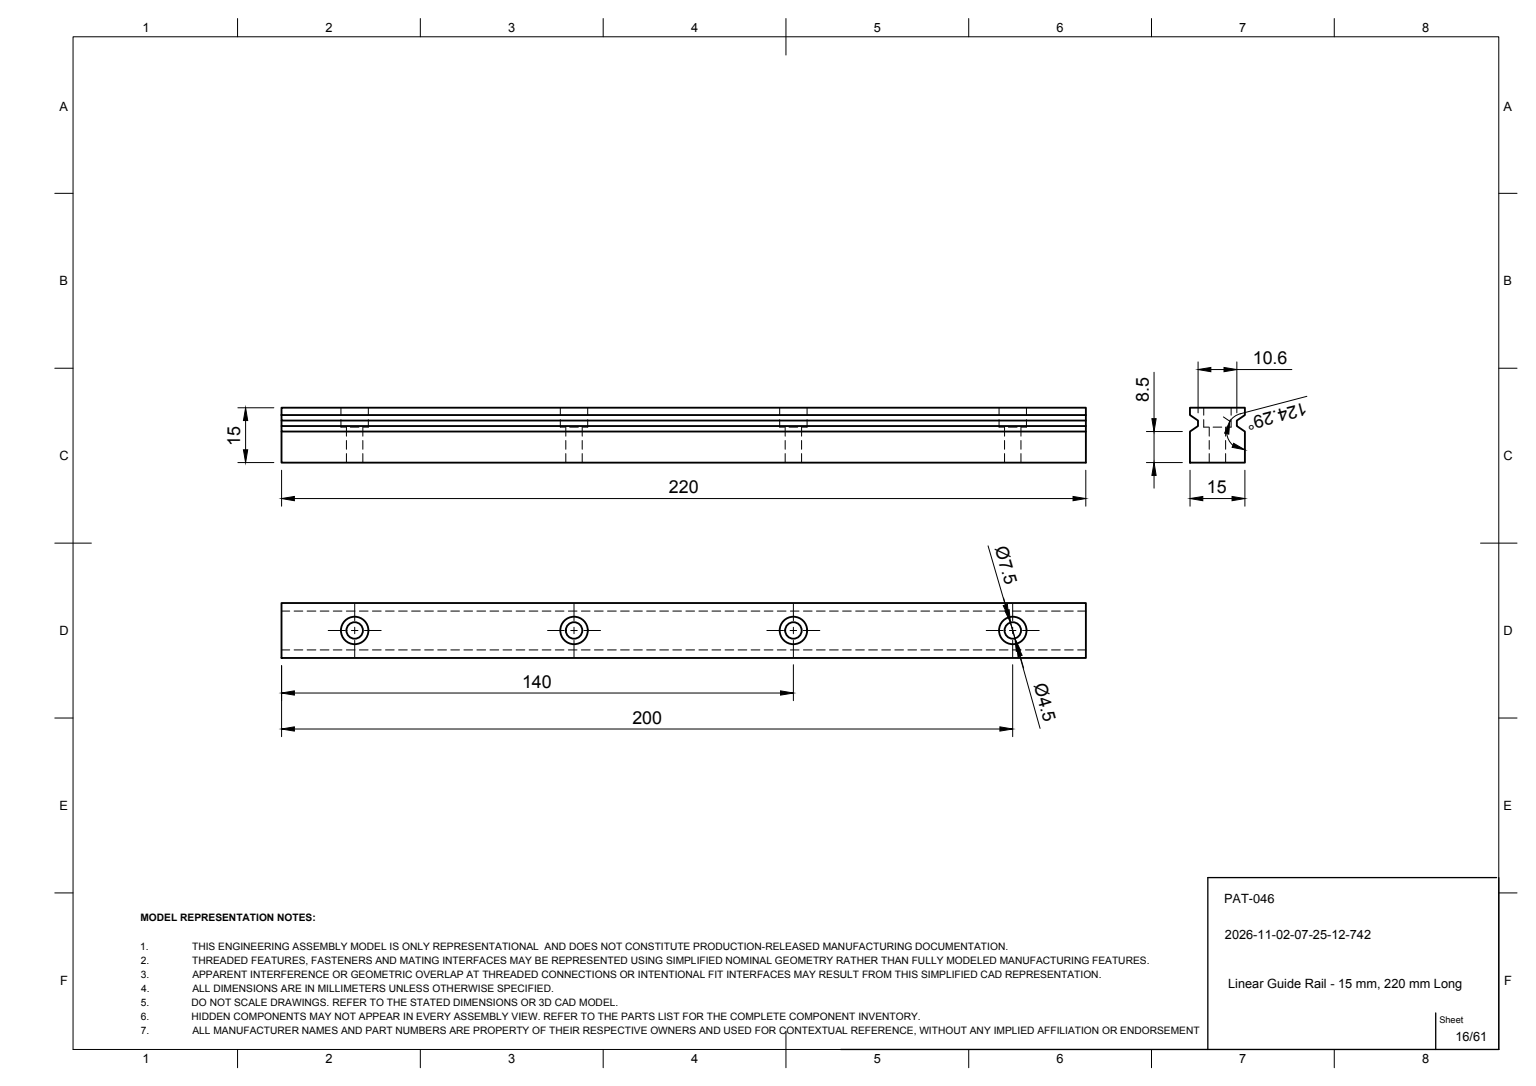
ISO-10303-21;
HEADER;
/* Generated by software containing ST-Developer
 * from STEP Tools, Inc. (www.steptools.com) 
 */

FILE_DESCRIPTION(
/* description */ ('Gear mesh backlash fixture'),
/* implementation_level */ '2;1');

FILE_NAME(
/* name */ 'Linear Guide Rail - 15 mm, 220 mm Long.step',
/* time_stamp */ '2026-10-28T03:26:00-07:00',
/* author */ (''),
/* organization */ (''),
/* preprocessor_version */ 'ST-DEVELOPER v20.2',
/* originating_system */ 'Autodesk Translation Framework v15.17.0.0',
/* authorisation */ '');

FILE_SCHEMA (('AUTOMOTIVE_DESIGN { 1 0 10303 214 3 1 1 }'));
ENDSEC;

DATA;
#10=MECHANICAL_DESIGN_GEOMETRIC_PRESENTATION_REPRESENTATION('',(#1027),#57900);
#927=SHAPE_REPRESENTATION_RELATIONSHIP('SRR','None',#58122,#977);
#977=ADVANCED_BREP_SHAPE_REPRESENTATION('',(#1092),#57855);
#1027=STYLED_ITEM('',(#58458),#1092);
#1092=MANIFOLD_SOLID_BREP('Body1',#13587);
#1205=FACE_BOUND('',#2643,.T.);
#1206=FACE_BOUND('',#2646,.T.);
#1207=FACE_BOUND('',#2649,.T.);
#1208=FACE_BOUND('',#2652,.T.);
#1209=FACE_BOUND('',#2662,.T.);
#1210=FACE_BOUND('',#2663,.T.);
#1211=FACE_BOUND('',#2664,.T.);
#1212=FACE_BOUND('',#2665,.T.);
#1213=FACE_BOUND('',#2672,.T.);
#1214=FACE_BOUND('',#2673,.T.);
#1215=FACE_BOUND('',#2674,.T.);
#1216=FACE_BOUND('',#2675,.T.);
#1395=PLANE('',#14457);
#1396=PLANE('',#14462);
#1397=PLANE('',#14467);
#1398=PLANE('',#14472);
#1399=PLANE('',#14482);
#1400=PLANE('',#14483);
#1401=PLANE('',#14484);
#1402=PLANE('',#14485);
#1403=PLANE('',#14486);
#1404=PLANE('',#14487);
#1405=PLANE('',#14488);
#1406=PLANE('',#14489);
#1407=PLANE('',#14490);
#1408=PLANE('',#14491);
#1409=PLANE('',#14492);
#1410=PLANE('',#14493);
#1411=PLANE('',#14494);
#1412=PLANE('',#14495);
#1814=FACE_OUTER_BOUND('',#2641,.T.);
#1815=FACE_OUTER_BOUND('',#2642,.T.);
#1816=FACE_OUTER_BOUND('',#2644,.T.);
#1817=FACE_OUTER_BOUND('',#2645,.T.);
#1818=FACE_OUTER_BOUND('',#2647,.T.);
#1819=FACE_OUTER_BOUND('',#2648,.T.);
#1820=FACE_OUTER_BOUND('',#2650,.T.);
#1821=FACE_OUTER_BOUND('',#2651,.T.);
#1822=FACE_OUTER_BOUND('',#2653,.T.);
#1823=FACE_OUTER_BOUND('',#2654,.T.);
#1824=FACE_OUTER_BOUND('',#2655,.T.);
#1825=FACE_OUTER_BOUND('',#2656,.T.);
#1826=FACE_OUTER_BOUND('',#2657,.T.);
#1827=FACE_OUTER_BOUND('',#2658,.T.);
#1828=FACE_OUTER_BOUND('',#2659,.T.);
#1829=FACE_OUTER_BOUND('',#2660,.T.);
#1830=FACE_OUTER_BOUND('',#2661,.T.);
#1831=FACE_OUTER_BOUND('',#2666,.T.);
#1832=FACE_OUTER_BOUND('',#2667,.T.);
#1833=FACE_OUTER_BOUND('',#2668,.T.);
#1834=FACE_OUTER_BOUND('',#2669,.T.);
#1835=FACE_OUTER_BOUND('',#2670,.T.);
#1836=FACE_OUTER_BOUND('',#2671,.T.);
#1837=FACE_OUTER_BOUND('',#2676,.T.);
#1838=FACE_OUTER_BOUND('',#2677,.T.);
#1839=FACE_OUTER_BOUND('',#2678,.T.);
#2641=EDGE_LOOP('',(#9427,#9428,#9429,#9430));
#2642=EDGE_LOOP('',(#9431));
#2643=EDGE_LOOP('',(#9432));
#2644=EDGE_LOOP('',(#9433,#9434,#9435,#9436));
#2645=EDGE_LOOP('',(#9437));
#2646=EDGE_LOOP('',(#9438));
#2647=EDGE_LOOP('',(#9439,#9440,#9441,#9442));
#2648=EDGE_LOOP('',(#9443));
#2649=EDGE_LOOP('',(#9444));
#2650=EDGE_LOOP('',(#9445,#9446,#9447,#9448));
#2651=EDGE_LOOP('',(#9449));
#2652=EDGE_LOOP('',(#9450));
#2653=EDGE_LOOP('',(#9451,#9452,#9453,#9454));
#2654=EDGE_LOOP('',(#9455,#9456,#9457,#9458));
#2655=EDGE_LOOP('',(#9459,#9460,#9461,#9462));
#2656=EDGE_LOOP('',(#9463,#9464,#9465,#9466));
#2657=EDGE_LOOP('',(#9467,#9468,#9469,#9470));
#2658=EDGE_LOOP('',(#9471,#9472,#9473,#9474));
#2659=EDGE_LOOP('',(#9475,#9476,#9477,#9478));
#2660=EDGE_LOOP('',(#9479,#9480,#9481,#9482));
#2661=EDGE_LOOP('',(#9483,#9484,#9485,#9486));
#2662=EDGE_LOOP('',(#9487));
#2663=EDGE_LOOP('',(#9488));
#2664=EDGE_LOOP('',(#9489));
#2665=EDGE_LOOP('',(#9490));
#2666=EDGE_LOOP('',(#9491,#9492,#9493,#9494));
#2667=EDGE_LOOP('',(#9495,#9496,#9497,#9498));
#2668=EDGE_LOOP('',(#9499,#9500,#9501,#9502));
#2669=EDGE_LOOP('',(#9503,#9504,#9505,#9506));
#2670=EDGE_LOOP('',(#9507,#9508,#9509,#9510));
#2671=EDGE_LOOP('',(#9511,#9512,#9513,#9514));
#2672=EDGE_LOOP('',(#9515));
#2673=EDGE_LOOP('',(#9516));
#2674=EDGE_LOOP('',(#9517));
#2675=EDGE_LOOP('',(#9518));
#2676=EDGE_LOOP('',(#9519,#9520,#9521,#9522));
#2677=EDGE_LOOP('',(#9523,#9524,#9525,#9526,#9527,#9528,#9529,#9530,#9531,
#9532,#9533,#9534));
#2678=EDGE_LOOP('',(#9535,#9536,#9537,#9538,#9539,#9540,#9541,#9542,#9543,
#9544,#9545,#9546));
#3553=LINE('',#19918,#4442);
#3554=LINE('',#19927,#4443);
#3555=LINE('',#19936,#4444);
#3556=LINE('',#19945,#4445);
#3557=LINE('',#19953,#4446);
#3558=LINE('',#19957,#4447);
#3559=LINE('',#19961,#4448);
#3560=LINE('',#19965,#4449);
#3561=LINE('',#19969,#4450);
#3562=LINE('',#19971,#4451);
#3563=LINE('',#19973,#4452);
#3564=LINE('',#19974,#4453);
#3565=LINE('',#19977,#4454);
#3566=LINE('',#19979,#4455);
#3567=LINE('',#19980,#4456);
#3568=LINE('',#19983,#4457);
#3569=LINE('',#19985,#4458);
#3570=LINE('',#19986,#4459);
#3571=LINE('',#19989,#4460);
#3572=LINE('',#19991,#4461);
#3573=LINE('',#19992,#4462);
#3574=LINE('',#19995,#4463);
#3575=LINE('',#19997,#4464);
#3576=LINE('',#19998,#4465);
#3577=LINE('',#20001,#4466);
#3578=LINE('',#20003,#4467);
#3579=LINE('',#20004,#4468);
#3580=LINE('',#20007,#4469);
#3581=LINE('',#20009,#4470);
#3582=LINE('',#20010,#4471);
#3583=LINE('',#20013,#4472);
#3584=LINE('',#20015,#4473);
#3585=LINE('',#20016,#4474);
#3586=LINE('',#20019,#4475);
#3587=LINE('',#20021,#4476);
#3588=LINE('',#20022,#4477);
#3589=LINE('',#20025,#4478);
#3590=LINE('',#20027,#4479);
#3591=LINE('',#20028,#4480);
#3592=LINE('',#20031,#4481);
#3593=LINE('',#20033,#4482);
#3594=LINE('',#20034,#4483);
#3595=LINE('',#20036,#4484);
#3596=LINE('',#20037,#4485);
#4442=VECTOR('',#16242,0.375);
#4443=VECTOR('',#16253,0.375);
#4444=VECTOR('',#16264,0.375);
#4445=VECTOR('',#16275,0.375);
#4446=VECTOR('',#16286,0.225);
#4447=VECTOR('',#16291,0.225);
#4448=VECTOR('',#16296,0.225);
#4449=VECTOR('',#16301,0.225000000000001);
#4450=VECTOR('',#16304,1.);
#4451=VECTOR('',#16305,1.);
#4452=VECTOR('',#16306,1.);
#4453=VECTOR('',#16307,1.);
#4454=VECTOR('',#16310,1.);
#4455=VECTOR('',#16311,1.);
#4456=VECTOR('',#16312,1.);
#4457=VECTOR('',#16315,1.);
#4458=VECTOR('',#16316,1.);
#4459=VECTOR('',#16317,1.);
#4460=VECTOR('',#16320,1.);
#4461=VECTOR('',#16321,1.);
#4462=VECTOR('',#16322,1.);
#4463=VECTOR('',#16325,1.);
#4464=VECTOR('',#16326,1.);
#4465=VECTOR('',#16327,1.);
#4466=VECTOR('',#16330,1.);
#4467=VECTOR('',#16331,1.);
#4468=VECTOR('',#16332,1.);
#4469=VECTOR('',#16335,1.);
#4470=VECTOR('',#16336,1.);
#4471=VECTOR('',#16337,1.);
#4472=VECTOR('',#16340,1.);
#4473=VECTOR('',#16341,1.);
#4474=VECTOR('',#16342,1.);
#4475=VECTOR('',#16345,1.);
#4476=VECTOR('',#16346,1.);
#4477=VECTOR('',#16347,1.);
#4478=VECTOR('',#16350,1.);
#4479=VECTOR('',#16351,1.);
#4480=VECTOR('',#16352,1.);
#4481=VECTOR('',#16355,1.);
#4482=VECTOR('',#16356,1.);
#4483=VECTOR('',#16357,1.);
#4484=VECTOR('',#16360,1.);
#4485=VECTOR('',#16361,1.);
#5314=CIRCLE('',#14455,0.375);
#5315=CIRCLE('',#14456,0.375);
#5316=CIRCLE('',#14458,0.225);
#5317=CIRCLE('',#14460,0.375);
#5318=CIRCLE('',#14461,0.375);
#5319=CIRCLE('',#14463,0.225);
#5320=CIRCLE('',#14465,0.375);
#5321=CIRCLE('',#14466,0.375);
#5322=CIRCLE('',#14468,0.225);
#5323=CIRCLE('',#14470,0.375);
#5324=CIRCLE('',#14471,0.375);
#5325=CIRCLE('',#14473,0.225000000000001);
#5326=CIRCLE('',#14475,0.225);
#5327=CIRCLE('',#14477,0.225);
#5328=CIRCLE('',#14479,0.225);
#5329=CIRCLE('',#14481,0.225000000000001);
#5959=VERTEX_POINT('',#19915);
#5960=VERTEX_POINT('',#19917);
#5961=VERTEX_POINT('',#19921);
#5962=VERTEX_POINT('',#19924);
#5963=VERTEX_POINT('',#19926);
#5964=VERTEX_POINT('',#19930);
#5965=VERTEX_POINT('',#19933);
#5966=VERTEX_POINT('',#19935);
#5967=VERTEX_POINT('',#19939);
#5968=VERTEX_POINT('',#19942);
#5969=VERTEX_POINT('',#19944);
#5970=VERTEX_POINT('',#19948);
#5971=VERTEX_POINT('',#19951);
#5972=VERTEX_POINT('',#19955);
#5973=VERTEX_POINT('',#19959);
#5974=VERTEX_POINT('',#19963);
#5975=VERTEX_POINT('',#19967);
#5976=VERTEX_POINT('',#19968);
#5977=VERTEX_POINT('',#19970);
#5978=VERTEX_POINT('',#19972);
#5979=VERTEX_POINT('',#19976);
#5980=VERTEX_POINT('',#19978);
#5981=VERTEX_POINT('',#19982);
#5982=VERTEX_POINT('',#19984);
#5983=VERTEX_POINT('',#19988);
#5984=VERTEX_POINT('',#19990);
#5985=VERTEX_POINT('',#19994);
#5986=VERTEX_POINT('',#19996);
#5987=VERTEX_POINT('',#20000);
#5988=VERTEX_POINT('',#20002);
#5989=VERTEX_POINT('',#20006);
#5990=VERTEX_POINT('',#20008);
#5991=VERTEX_POINT('',#20012);
#5992=VERTEX_POINT('',#20014);
#5993=VERTEX_POINT('',#20018);
#5994=VERTEX_POINT('',#20020);
#5995=VERTEX_POINT('',#20024);
#5996=VERTEX_POINT('',#20026);
#5997=VERTEX_POINT('',#20030);
#5998=VERTEX_POINT('',#20032);
#7300=EDGE_CURVE('',#5959,#5959,#5314,.T.);
#7301=EDGE_CURVE('',#5959,#5960,#3553,.T.);
#7302=EDGE_CURVE('',#5960,#5960,#5315,.T.);
#7303=EDGE_CURVE('',#5961,#5961,#5316,.T.);
#7304=EDGE_CURVE('',#5962,#5962,#5317,.T.);
#7305=EDGE_CURVE('',#5962,#5963,#3554,.T.);
#7306=EDGE_CURVE('',#5963,#5963,#5318,.T.);
#7307=EDGE_CURVE('',#5964,#5964,#5319,.T.);
#7308=EDGE_CURVE('',#5965,#5965,#5320,.T.);
#7309=EDGE_CURVE('',#5965,#5966,#3555,.T.);
#7310=EDGE_CURVE('',#5966,#5966,#5321,.T.);
#7311=EDGE_CURVE('',#5967,#5967,#5322,.T.);
#7312=EDGE_CURVE('',#5968,#5968,#5323,.T.);
#7313=EDGE_CURVE('',#5968,#5969,#3556,.T.);
#7314=EDGE_CURVE('',#5969,#5969,#5324,.T.);
#7315=EDGE_CURVE('',#5970,#5970,#5325,.T.);
#7316=EDGE_CURVE('',#5971,#5971,#5326,.T.);
#7317=EDGE_CURVE('',#5971,#5961,#3557,.T.);
#7318=EDGE_CURVE('',#5972,#5972,#5327,.T.);
#7319=EDGE_CURVE('',#5972,#5964,#3558,.T.);
#7320=EDGE_CURVE('',#5973,#5973,#5328,.T.);
#7321=EDGE_CURVE('',#5973,#5967,#3559,.T.);
#7322=EDGE_CURVE('',#5974,#5974,#5329,.T.);
#7323=EDGE_CURVE('',#5974,#5970,#3560,.T.);
#7324=EDGE_CURVE('',#5975,#5976,#3561,.T.);
#7325=EDGE_CURVE('',#5976,#5977,#3562,.T.);
#7326=EDGE_CURVE('',#5978,#5977,#3563,.T.);
#7327=EDGE_CURVE('',#5975,#5978,#3564,.T.);
#7328=EDGE_CURVE('',#5979,#5975,#3565,.T.);
#7329=EDGE_CURVE('',#5980,#5978,#3566,.T.);
#7330=EDGE_CURVE('',#5979,#5980,#3567,.T.);
#7331=EDGE_CURVE('',#5981,#5979,#3568,.T.);
#7332=EDGE_CURVE('',#5982,#5980,#3569,.T.);
#7333=EDGE_CURVE('',#5981,#5982,#3570,.T.);
#7334=EDGE_CURVE('',#5983,#5981,#3571,.T.);
#7335=EDGE_CURVE('',#5984,#5982,#3572,.T.);
#7336=EDGE_CURVE('',#5983,#5984,#3573,.T.);
#7337=EDGE_CURVE('',#5985,#5983,#3574,.T.);
#7338=EDGE_CURVE('',#5986,#5984,#3575,.T.);
#7339=EDGE_CURVE('',#5985,#5986,#3576,.T.);
#7340=EDGE_CURVE('',#5987,#5985,#3577,.T.);
#7341=EDGE_CURVE('',#5988,#5986,#3578,.T.);
#7342=EDGE_CURVE('',#5987,#5988,#3579,.T.);
#7343=EDGE_CURVE('',#5989,#5987,#3580,.T.);
#7344=EDGE_CURVE('',#5990,#5988,#3581,.T.);
#7345=EDGE_CURVE('',#5989,#5990,#3582,.T.);
#7346=EDGE_CURVE('',#5991,#5989,#3583,.T.);
#7347=EDGE_CURVE('',#5992,#5990,#3584,.T.);
#7348=EDGE_CURVE('',#5991,#5992,#3585,.T.);
#7349=EDGE_CURVE('',#5993,#5991,#3586,.T.);
#7350=EDGE_CURVE('',#5994,#5992,#3587,.T.);
#7351=EDGE_CURVE('',#5993,#5994,#3588,.T.);
#7352=EDGE_CURVE('',#5995,#5993,#3589,.T.);
#7353=EDGE_CURVE('',#5996,#5994,#3590,.T.);
#7354=EDGE_CURVE('',#5995,#5996,#3591,.T.);
#7355=EDGE_CURVE('',#5997,#5995,#3592,.T.);
#7356=EDGE_CURVE('',#5998,#5996,#3593,.T.);
#7357=EDGE_CURVE('',#5997,#5998,#3594,.T.);
#7358=EDGE_CURVE('',#5976,#5997,#3595,.T.);
#7359=EDGE_CURVE('',#5977,#5998,#3596,.T.);
#9427=ORIENTED_EDGE('',*,*,#7300,.F.);
#9428=ORIENTED_EDGE('',*,*,#7301,.T.);
#9429=ORIENTED_EDGE('',*,*,#7302,.F.);
#9430=ORIENTED_EDGE('',*,*,#7301,.F.);
#9431=ORIENTED_EDGE('',*,*,#7300,.T.);
#9432=ORIENTED_EDGE('',*,*,#7303,.F.);
#9433=ORIENTED_EDGE('',*,*,#7304,.F.);
#9434=ORIENTED_EDGE('',*,*,#7305,.T.);
#9435=ORIENTED_EDGE('',*,*,#7306,.F.);
#9436=ORIENTED_EDGE('',*,*,#7305,.F.);
#9437=ORIENTED_EDGE('',*,*,#7304,.T.);
#9438=ORIENTED_EDGE('',*,*,#7307,.F.);
#9439=ORIENTED_EDGE('',*,*,#7308,.F.);
#9440=ORIENTED_EDGE('',*,*,#7309,.T.);
#9441=ORIENTED_EDGE('',*,*,#7310,.F.);
#9442=ORIENTED_EDGE('',*,*,#7309,.F.);
#9443=ORIENTED_EDGE('',*,*,#7308,.T.);
#9444=ORIENTED_EDGE('',*,*,#7311,.F.);
#9445=ORIENTED_EDGE('',*,*,#7312,.F.);
#9446=ORIENTED_EDGE('',*,*,#7313,.T.);
#9447=ORIENTED_EDGE('',*,*,#7314,.F.);
#9448=ORIENTED_EDGE('',*,*,#7313,.F.);
#9449=ORIENTED_EDGE('',*,*,#7312,.T.);
#9450=ORIENTED_EDGE('',*,*,#7315,.F.);
#9451=ORIENTED_EDGE('',*,*,#7316,.F.);
#9452=ORIENTED_EDGE('',*,*,#7317,.T.);
#9453=ORIENTED_EDGE('',*,*,#7303,.T.);
#9454=ORIENTED_EDGE('',*,*,#7317,.F.);
#9455=ORIENTED_EDGE('',*,*,#7318,.F.);
#9456=ORIENTED_EDGE('',*,*,#7319,.T.);
#9457=ORIENTED_EDGE('',*,*,#7307,.T.);
#9458=ORIENTED_EDGE('',*,*,#7319,.F.);
#9459=ORIENTED_EDGE('',*,*,#7320,.F.);
#9460=ORIENTED_EDGE('',*,*,#7321,.T.);
#9461=ORIENTED_EDGE('',*,*,#7311,.T.);
#9462=ORIENTED_EDGE('',*,*,#7321,.F.);
#9463=ORIENTED_EDGE('',*,*,#7322,.F.);
#9464=ORIENTED_EDGE('',*,*,#7323,.T.);
#9465=ORIENTED_EDGE('',*,*,#7315,.T.);
#9466=ORIENTED_EDGE('',*,*,#7323,.F.);
#9467=ORIENTED_EDGE('',*,*,#7324,.T.);
#9468=ORIENTED_EDGE('',*,*,#7325,.T.);
#9469=ORIENTED_EDGE('',*,*,#7326,.F.);
#9470=ORIENTED_EDGE('',*,*,#7327,.F.);
#9471=ORIENTED_EDGE('',*,*,#7328,.T.);
#9472=ORIENTED_EDGE('',*,*,#7327,.T.);
#9473=ORIENTED_EDGE('',*,*,#7329,.F.);
#9474=ORIENTED_EDGE('',*,*,#7330,.F.);
#9475=ORIENTED_EDGE('',*,*,#7331,.T.);
#9476=ORIENTED_EDGE('',*,*,#7330,.T.);
#9477=ORIENTED_EDGE('',*,*,#7332,.F.);
#9478=ORIENTED_EDGE('',*,*,#7333,.F.);
#9479=ORIENTED_EDGE('',*,*,#7334,.T.);
#9480=ORIENTED_EDGE('',*,*,#7333,.T.);
#9481=ORIENTED_EDGE('',*,*,#7335,.F.);
#9482=ORIENTED_EDGE('',*,*,#7336,.F.);
#9483=ORIENTED_EDGE('',*,*,#7337,.T.);
#9484=ORIENTED_EDGE('',*,*,#7336,.T.);
#9485=ORIENTED_EDGE('',*,*,#7338,.F.);
#9486=ORIENTED_EDGE('',*,*,#7339,.F.);
#9487=ORIENTED_EDGE('',*,*,#7314,.T.);
#9488=ORIENTED_EDGE('',*,*,#7310,.T.);
#9489=ORIENTED_EDGE('',*,*,#7306,.T.);
#9490=ORIENTED_EDGE('',*,*,#7302,.T.);
#9491=ORIENTED_EDGE('',*,*,#7340,.T.);
#9492=ORIENTED_EDGE('',*,*,#7339,.T.);
#9493=ORIENTED_EDGE('',*,*,#7341,.F.);
#9494=ORIENTED_EDGE('',*,*,#7342,.F.);
#9495=ORIENTED_EDGE('',*,*,#7343,.T.);
#9496=ORIENTED_EDGE('',*,*,#7342,.T.);
#9497=ORIENTED_EDGE('',*,*,#7344,.F.);
#9498=ORIENTED_EDGE('',*,*,#7345,.F.);
#9499=ORIENTED_EDGE('',*,*,#7346,.T.);
#9500=ORIENTED_EDGE('',*,*,#7345,.T.);
#9501=ORIENTED_EDGE('',*,*,#7347,.F.);
#9502=ORIENTED_EDGE('',*,*,#7348,.F.);
#9503=ORIENTED_EDGE('',*,*,#7349,.T.);
#9504=ORIENTED_EDGE('',*,*,#7348,.T.);
#9505=ORIENTED_EDGE('',*,*,#7350,.F.);
#9506=ORIENTED_EDGE('',*,*,#7351,.F.);
#9507=ORIENTED_EDGE('',*,*,#7352,.T.);
#9508=ORIENTED_EDGE('',*,*,#7351,.T.);
#9509=ORIENTED_EDGE('',*,*,#7353,.F.);
#9510=ORIENTED_EDGE('',*,*,#7354,.F.);
#9511=ORIENTED_EDGE('',*,*,#7355,.T.);
#9512=ORIENTED_EDGE('',*,*,#7354,.T.);
#9513=ORIENTED_EDGE('',*,*,#7356,.F.);
#9514=ORIENTED_EDGE('',*,*,#7357,.F.);
#9515=ORIENTED_EDGE('',*,*,#7316,.T.);
#9516=ORIENTED_EDGE('',*,*,#7318,.T.);
#9517=ORIENTED_EDGE('',*,*,#7320,.T.);
#9518=ORIENTED_EDGE('',*,*,#7322,.T.);
#9519=ORIENTED_EDGE('',*,*,#7358,.T.);
#9520=ORIENTED_EDGE('',*,*,#7357,.T.);
#9521=ORIENTED_EDGE('',*,*,#7359,.F.);
#9522=ORIENTED_EDGE('',*,*,#7325,.F.);
#9523=ORIENTED_EDGE('',*,*,#7359,.T.);
#9524=ORIENTED_EDGE('',*,*,#7356,.T.);
#9525=ORIENTED_EDGE('',*,*,#7353,.T.);
#9526=ORIENTED_EDGE('',*,*,#7350,.T.);
#9527=ORIENTED_EDGE('',*,*,#7347,.T.);
#9528=ORIENTED_EDGE('',*,*,#7344,.T.);
#9529=ORIENTED_EDGE('',*,*,#7341,.T.);
#9530=ORIENTED_EDGE('',*,*,#7338,.T.);
#9531=ORIENTED_EDGE('',*,*,#7335,.T.);
#9532=ORIENTED_EDGE('',*,*,#7332,.T.);
#9533=ORIENTED_EDGE('',*,*,#7329,.T.);
#9534=ORIENTED_EDGE('',*,*,#7326,.T.);
#9535=ORIENTED_EDGE('',*,*,#7358,.F.);
#9536=ORIENTED_EDGE('',*,*,#7324,.F.);
#9537=ORIENTED_EDGE('',*,*,#7328,.F.);
#9538=ORIENTED_EDGE('',*,*,#7331,.F.);
#9539=ORIENTED_EDGE('',*,*,#7334,.F.);
#9540=ORIENTED_EDGE('',*,*,#7337,.F.);
#9541=ORIENTED_EDGE('',*,*,#7340,.F.);
#9542=ORIENTED_EDGE('',*,*,#7343,.F.);
#9543=ORIENTED_EDGE('',*,*,#7346,.F.);
#9544=ORIENTED_EDGE('',*,*,#7349,.F.);
#9545=ORIENTED_EDGE('',*,*,#7352,.F.);
#9546=ORIENTED_EDGE('',*,*,#7355,.F.);
#12640=CYLINDRICAL_SURFACE('',#14454,0.375);
#12641=CYLINDRICAL_SURFACE('',#14459,0.375);
#12642=CYLINDRICAL_SURFACE('',#14464,0.375);
#12643=CYLINDRICAL_SURFACE('',#14469,0.375);
#12644=CYLINDRICAL_SURFACE('',#14474,0.225);
#12645=CYLINDRICAL_SURFACE('',#14476,0.225);
#12646=CYLINDRICAL_SURFACE('',#14478,0.225);
#12647=CYLINDRICAL_SURFACE('',#14480,0.225000000000001);
#12931=ADVANCED_FACE('',(#1814),#12640,.F.);
#12932=ADVANCED_FACE('',(#1815,#1205),#1395,.T.);
#12933=ADVANCED_FACE('',(#1816),#12641,.F.);
#12934=ADVANCED_FACE('',(#1817,#1206),#1396,.T.);
#12935=ADVANCED_FACE('',(#1818),#12642,.F.);
#12936=ADVANCED_FACE('',(#1819,#1207),#1397,.T.);
#12937=ADVANCED_FACE('',(#1820),#12643,.F.);
#12938=ADVANCED_FACE('',(#1821,#1208),#1398,.T.);
#12939=ADVANCED_FACE('',(#1822),#12644,.F.);
#12940=ADVANCED_FACE('',(#1823),#12645,.F.);
#12941=ADVANCED_FACE('',(#1824),#12646,.F.);
#12942=ADVANCED_FACE('',(#1825),#12647,.F.);
#12943=ADVANCED_FACE('',(#1826),#1399,.T.);
#12944=ADVANCED_FACE('',(#1827),#1400,.T.);
#12945=ADVANCED_FACE('',(#1828),#1401,.T.);
#12946=ADVANCED_FACE('',(#1829),#1402,.T.);
#12947=ADVANCED_FACE('',(#1830,#1209,#1210,#1211,#1212),#1403,.T.);
#12948=ADVANCED_FACE('',(#1831),#1404,.T.);
#12949=ADVANCED_FACE('',(#1832),#1405,.T.);
#12950=ADVANCED_FACE('',(#1833),#1406,.T.);
#12951=ADVANCED_FACE('',(#1834),#1407,.T.);
#12952=ADVANCED_FACE('',(#1835),#1408,.T.);
#12953=ADVANCED_FACE('',(#1836,#1213,#1214,#1215,#1216),#1409,.T.);
#12954=ADVANCED_FACE('',(#1837),#1410,.T.);
#12955=ADVANCED_FACE('',(#1838),#1411,.T.);
#12956=ADVANCED_FACE('',(#1839),#1412,.F.);
#13587=CLOSED_SHELL('',(#12931,#12932,#12933,#12934,#12935,#12936,#12937,
#12938,#12939,#12940,#12941,#12942,#12943,#12944,#12945,#12946,#12947,#12948,
#12949,#12950,#12951,#12952,#12953,#12954,#12955,#12956));
#14453=AXIS2_PLACEMENT_3D('',#19913,#16236,#16237);
#14454=AXIS2_PLACEMENT_3D('',#19914,#16238,#16239);
#14455=AXIS2_PLACEMENT_3D('',#19916,#16240,#16241);
#14456=AXIS2_PLACEMENT_3D('',#19919,#16243,#16244);
#14457=AXIS2_PLACEMENT_3D('',#19920,#16245,#16246);
#14458=AXIS2_PLACEMENT_3D('',#19922,#16247,#16248);
#14459=AXIS2_PLACEMENT_3D('',#19923,#16249,#16250);
#14460=AXIS2_PLACEMENT_3D('',#19925,#16251,#16252);
#14461=AXIS2_PLACEMENT_3D('',#19928,#16254,#16255);
#14462=AXIS2_PLACEMENT_3D('',#19929,#16256,#16257);
#14463=AXIS2_PLACEMENT_3D('',#19931,#16258,#16259);
#14464=AXIS2_PLACEMENT_3D('',#19932,#16260,#16261);
#14465=AXIS2_PLACEMENT_3D('',#19934,#16262,#16263);
#14466=AXIS2_PLACEMENT_3D('',#19937,#16265,#16266);
#14467=AXIS2_PLACEMENT_3D('',#19938,#16267,#16268);
#14468=AXIS2_PLACEMENT_3D('',#19940,#16269,#16270);
#14469=AXIS2_PLACEMENT_3D('',#19941,#16271,#16272);
#14470=AXIS2_PLACEMENT_3D('',#19943,#16273,#16274);
#14471=AXIS2_PLACEMENT_3D('',#19946,#16276,#16277);
#14472=AXIS2_PLACEMENT_3D('',#19947,#16278,#16279);
#14473=AXIS2_PLACEMENT_3D('',#19949,#16280,#16281);
#14474=AXIS2_PLACEMENT_3D('',#19950,#16282,#16283);
#14475=AXIS2_PLACEMENT_3D('',#19952,#16284,#16285);
#14476=AXIS2_PLACEMENT_3D('',#19954,#16287,#16288);
#14477=AXIS2_PLACEMENT_3D('',#19956,#16289,#16290);
#14478=AXIS2_PLACEMENT_3D('',#19958,#16292,#16293);
#14479=AXIS2_PLACEMENT_3D('',#19960,#16294,#16295);
#14480=AXIS2_PLACEMENT_3D('',#19962,#16297,#16298);
#14481=AXIS2_PLACEMENT_3D('',#19964,#16299,#16300);
#14482=AXIS2_PLACEMENT_3D('',#19966,#16302,#16303);
#14483=AXIS2_PLACEMENT_3D('',#19975,#16308,#16309);
#14484=AXIS2_PLACEMENT_3D('',#19981,#16313,#16314);
#14485=AXIS2_PLACEMENT_3D('',#19987,#16318,#16319);
#14486=AXIS2_PLACEMENT_3D('',#19993,#16323,#16324);
#14487=AXIS2_PLACEMENT_3D('',#19999,#16328,#16329);
#14488=AXIS2_PLACEMENT_3D('',#20005,#16333,#16334);
#14489=AXIS2_PLACEMENT_3D('',#20011,#16338,#16339);
#14490=AXIS2_PLACEMENT_3D('',#20017,#16343,#16344);
#14491=AXIS2_PLACEMENT_3D('',#20023,#16348,#16349);
#14492=AXIS2_PLACEMENT_3D('',#20029,#16353,#16354);
#14493=AXIS2_PLACEMENT_3D('',#20035,#16358,#16359);
#14494=AXIS2_PLACEMENT_3D('',#20038,#16362,#16363);
#14495=AXIS2_PLACEMENT_3D('',#20039,#16364,#16365);
#16236=DIRECTION('axis',(0.,0.,1.));
#16237=DIRECTION('refdir',(1.,0.,0.));
#16238=DIRECTION('center_axis',(0.,0.,1.));
#16239=DIRECTION('ref_axis',(1.,0.,0.));
#16240=DIRECTION('center_axis',(0.,0.,1.));
#16241=DIRECTION('ref_axis',(1.,0.,0.));
#16242=DIRECTION('',(0.,0.,1.));
#16243=DIRECTION('center_axis',(0.,0.,-1.));
#16244=DIRECTION('ref_axis',(1.,0.,0.));
#16245=DIRECTION('center_axis',(0.,0.,1.));
#16246=DIRECTION('ref_axis',(1.,0.,0.));
#16247=DIRECTION('center_axis',(0.,0.,1.));
#16248=DIRECTION('ref_axis',(1.,0.,0.));
#16249=DIRECTION('center_axis',(0.,0.,1.));
#16250=DIRECTION('ref_axis',(1.,0.,0.));
#16251=DIRECTION('center_axis',(0.,0.,1.));
#16252=DIRECTION('ref_axis',(1.,0.,0.));
#16253=DIRECTION('',(0.,0.,1.));
#16254=DIRECTION('center_axis',(0.,0.,-1.));
#16255=DIRECTION('ref_axis',(1.,0.,0.));
#16256=DIRECTION('center_axis',(0.,0.,1.));
#16257=DIRECTION('ref_axis',(1.,0.,0.));
#16258=DIRECTION('center_axis',(0.,0.,1.));
#16259=DIRECTION('ref_axis',(1.,0.,0.));
#16260=DIRECTION('center_axis',(0.,0.,1.));
#16261=DIRECTION('ref_axis',(1.,0.,0.));
#16262=DIRECTION('center_axis',(0.,0.,1.));
#16263=DIRECTION('ref_axis',(1.,0.,0.));
#16264=DIRECTION('',(0.,0.,1.));
#16265=DIRECTION('center_axis',(0.,0.,-1.));
#16266=DIRECTION('ref_axis',(1.,0.,0.));
#16267=DIRECTION('center_axis',(0.,0.,1.));
#16268=DIRECTION('ref_axis',(1.,0.,0.));
#16269=DIRECTION('center_axis',(0.,0.,1.));
#16270=DIRECTION('ref_axis',(1.,0.,0.));
#16271=DIRECTION('center_axis',(0.,0.,1.));
#16272=DIRECTION('ref_axis',(1.,0.,0.));
#16273=DIRECTION('center_axis',(0.,0.,1.));
#16274=DIRECTION('ref_axis',(1.,0.,0.));
#16275=DIRECTION('',(0.,0.,1.));
#16276=DIRECTION('center_axis',(0.,0.,-1.));
#16277=DIRECTION('ref_axis',(1.,0.,0.));
#16278=DIRECTION('center_axis',(0.,0.,1.));
#16279=DIRECTION('ref_axis',(1.,0.,0.));
#16280=DIRECTION('center_axis',(0.,0.,1.));
#16281=DIRECTION('ref_axis',(1.,0.,0.));
#16282=DIRECTION('center_axis',(0.,0.,1.));
#16283=DIRECTION('ref_axis',(1.,0.,0.));
#16284=DIRECTION('center_axis',(0.,0.,1.));
#16285=DIRECTION('ref_axis',(1.,0.,0.));
#16286=DIRECTION('',(0.,0.,1.));
#16287=DIRECTION('center_axis',(0.,0.,1.));
#16288=DIRECTION('ref_axis',(1.,0.,0.));
#16289=DIRECTION('center_axis',(0.,0.,1.));
#16290=DIRECTION('ref_axis',(1.,0.,0.));
#16291=DIRECTION('',(0.,0.,1.));
#16292=DIRECTION('center_axis',(0.,0.,1.));
#16293=DIRECTION('ref_axis',(1.,0.,0.));
#16294=DIRECTION('center_axis',(0.,0.,1.));
#16295=DIRECTION('ref_axis',(1.,0.,0.));
#16296=DIRECTION('',(0.,0.,1.));
#16297=DIRECTION('center_axis',(0.,0.,1.));
#16298=DIRECTION('ref_axis',(1.,0.,0.));
#16299=DIRECTION('center_axis',(0.,0.,1.));
#16300=DIRECTION('ref_axis',(1.,0.,0.));
#16301=DIRECTION('',(0.,0.,1.));
#16302=DIRECTION('center_axis',(0.,-0.56333682464151,0.826227342807548));
#16303=DIRECTION('ref_axis',(0.,-0.826227342807548,-0.56333682464151));
#16304=DIRECTION('',(0.,-0.826227342807548,-0.56333682464151));
#16305=DIRECTION('',(1.,0.,0.));
#16306=DIRECTION('',(0.,-0.826227342807548,-0.56333682464151));
#16307=DIRECTION('',(1.,0.,0.));
#16308=DIRECTION('center_axis',(0.,-1.,0.));
#16309=DIRECTION('ref_axis',(0.,0.,-1.));
#16310=DIRECTION('',(0.,0.,-1.));
#16311=DIRECTION('',(0.,0.,-1.));
#16312=DIRECTION('',(1.,0.,0.));
#16313=DIRECTION('center_axis',(0.,-0.56333682464151,-0.826227342807548));
#16314=DIRECTION('ref_axis',(0.,0.826227342807548,-0.56333682464151));
#16315=DIRECTION('',(0.,0.826227342807548,-0.56333682464151));
#16316=DIRECTION('',(0.,0.826227342807548,-0.56333682464151));
#16317=DIRECTION('',(1.,0.,0.));
#16318=DIRECTION('center_axis',(0.,-1.,0.));
#16319=DIRECTION('ref_axis',(0.,0.,-1.));
#16320=DIRECTION('',(0.,0.,-1.));
#16321=DIRECTION('',(0.,0.,-1.));
#16322=DIRECTION('',(1.,0.,0.));
#16323=DIRECTION('center_axis',(0.,0.,1.));
#16324=DIRECTION('ref_axis',(0.,-1.,0.));
#16325=DIRECTION('',(0.,-1.,0.));
#16326=DIRECTION('',(0.,-1.,0.));
#16327=DIRECTION('',(1.,0.,0.));
#16328=DIRECTION('center_axis',(0.,1.,0.));
#16329=DIRECTION('ref_axis',(0.,0.,1.));
#16330=DIRECTION('',(0.,0.,1.));
#16331=DIRECTION('',(0.,0.,1.));
#16332=DIRECTION('',(1.,0.,0.));
#16333=DIRECTION('center_axis',(0.,0.56333682464151,-0.826227342807548));
#16334=DIRECTION('ref_axis',(0.,0.826227342807548,0.56333682464151));
#16335=DIRECTION('',(0.,0.826227342807548,0.56333682464151));
#16336=DIRECTION('',(0.,0.826227342807548,0.56333682464151));
#16337=DIRECTION('',(1.,0.,0.));
#16338=DIRECTION('center_axis',(0.,1.,0.));
#16339=DIRECTION('ref_axis',(0.,0.,1.));
#16340=DIRECTION('',(0.,0.,1.));
#16341=DIRECTION('',(0.,0.,1.));
#16342=DIRECTION('',(1.,0.,0.));
#16343=DIRECTION('center_axis',(0.,0.56333682464151,0.826227342807548));
#16344=DIRECTION('ref_axis',(0.,-0.826227342807548,0.56333682464151));
#16345=DIRECTION('',(0.,-0.826227342807548,0.56333682464151));
#16346=DIRECTION('',(0.,-0.826227342807548,0.56333682464151));
#16347=DIRECTION('',(1.,0.,0.));
#16348=DIRECTION('center_axis',(0.,1.,0.));
#16349=DIRECTION('ref_axis',(0.,0.,1.));
#16350=DIRECTION('',(0.,0.,1.));
#16351=DIRECTION('',(0.,0.,1.));
#16352=DIRECTION('',(1.,0.,0.));
#16353=DIRECTION('center_axis',(0.,0.,-1.));
#16354=DIRECTION('ref_axis',(0.,1.,0.));
#16355=DIRECTION('',(0.,1.,0.));
#16356=DIRECTION('',(0.,1.,0.));
#16357=DIRECTION('',(1.,0.,0.));
#16358=DIRECTION('center_axis',(0.,-1.,0.));
#16359=DIRECTION('ref_axis',(0.,0.,-1.));
#16360=DIRECTION('',(0.,0.,-1.));
#16361=DIRECTION('',(0.,0.,-1.));
#16362=DIRECTION('center_axis',(1.,0.,0.));
#16363=DIRECTION('ref_axis',(0.,0.,-1.));
#16364=DIRECTION('center_axis',(1.,0.,0.));
#16365=DIRECTION('ref_axis',(0.,0.,-1.));
#19913=CARTESIAN_POINT('',(0.,0.,0.));
#19914=CARTESIAN_POINT('Origin',(14.,0.,0.97));
#19915=CARTESIAN_POINT('',(13.625,-4.59242549680257E-17,0.97));
#19916=CARTESIAN_POINT('Origin',(14.,0.,0.97));
#19917=CARTESIAN_POINT('',(13.625,4.59242549680257E-17,1.5));
#19918=CARTESIAN_POINT('',(13.625,-4.59242549680257E-17,0.97));
#19919=CARTESIAN_POINT('Origin',(14.,0.,1.5));
#19920=CARTESIAN_POINT('Origin',(14.,0.,0.97));
#19921=CARTESIAN_POINT('',(13.775,-2.75545529808154E-17,0.97));
#19922=CARTESIAN_POINT('Origin',(14.,0.,0.97));
#19923=CARTESIAN_POINT('Origin',(8.,0.,0.97));
#19924=CARTESIAN_POINT('',(7.625,-4.59242549680257E-17,0.97));
#19925=CARTESIAN_POINT('Origin',(8.,0.,0.97));
#19926=CARTESIAN_POINT('',(7.625,4.59242549680257E-17,1.5));
#19927=CARTESIAN_POINT('',(7.625,-4.59242549680257E-17,0.97));
#19928=CARTESIAN_POINT('Origin',(8.,0.,1.5));
#19929=CARTESIAN_POINT('Origin',(8.,0.,0.97));
#19930=CARTESIAN_POINT('',(7.775,-2.75545529808154E-17,0.97));
#19931=CARTESIAN_POINT('Origin',(8.,0.,0.97));
#19932=CARTESIAN_POINT('Origin',(2.,0.,0.97));
#19933=CARTESIAN_POINT('',(1.625,-4.59242549680257E-17,0.97));
#19934=CARTESIAN_POINT('Origin',(2.,0.,0.97));
#19935=CARTESIAN_POINT('',(1.625,4.59242549680257E-17,1.5));
#19936=CARTESIAN_POINT('',(1.625,-4.59242549680257E-17,0.97));
#19937=CARTESIAN_POINT('Origin',(2.,0.,1.5));
#19938=CARTESIAN_POINT('Origin',(2.,0.,0.97));
#19939=CARTESIAN_POINT('',(1.775,-2.75545529808155E-17,0.97));
#19940=CARTESIAN_POINT('Origin',(2.,0.,0.97));
#19941=CARTESIAN_POINT('Origin',(20.,0.,0.97));
#19942=CARTESIAN_POINT('',(19.625,-4.59242549680257E-17,0.97));
#19943=CARTESIAN_POINT('Origin',(20.,0.,0.97));
#19944=CARTESIAN_POINT('',(19.625,4.59242549680257E-17,1.5));
#19945=CARTESIAN_POINT('',(19.625,-4.59242549680257E-17,0.97));
#19946=CARTESIAN_POINT('Origin',(20.,0.,1.5));
#19947=CARTESIAN_POINT('Origin',(20.,0.,0.97));
#19948=CARTESIAN_POINT('',(19.775,-2.75545529808156E-17,0.97));
#19949=CARTESIAN_POINT('Origin',(20.,0.,0.97));
#19950=CARTESIAN_POINT('Origin',(14.,0.,-0.1));
#19951=CARTESIAN_POINT('',(13.775,-2.75545529808154E-17,0.));
#19952=CARTESIAN_POINT('Origin',(14.,0.,0.));
#19953=CARTESIAN_POINT('',(13.775,-2.75545529808154E-17,-0.1));
#19954=CARTESIAN_POINT('Origin',(8.,0.,-0.1));
#19955=CARTESIAN_POINT('',(7.775,-2.75545529808154E-17,0.));
#19956=CARTESIAN_POINT('Origin',(8.,0.,0.));
#19957=CARTESIAN_POINT('',(7.775,-2.75545529808154E-17,-0.1));
#19958=CARTESIAN_POINT('Origin',(2.,0.,-0.1));
#19959=CARTESIAN_POINT('',(1.775,-2.75545529808155E-17,0.));
#19960=CARTESIAN_POINT('Origin',(2.,0.,0.));
#19961=CARTESIAN_POINT('',(1.775,-2.75545529808155E-17,-0.1));
#19962=CARTESIAN_POINT('Origin',(20.,0.,-0.1));
#19963=CARTESIAN_POINT('',(19.775,-2.75545529808156E-17,0.));
#19964=CARTESIAN_POINT('Origin',(20.,0.,0.));
#19965=CARTESIAN_POINT('',(19.775,-2.75545529808156E-17,-0.1));
#19966=CARTESIAN_POINT('Origin',(0.,-0.53,1.));
#19967=CARTESIAN_POINT('',(0.,-0.53,1.));
#19968=CARTESIAN_POINT('',(0.,-0.75,0.85));
#19969=CARTESIAN_POINT('',(0.,-0.53,1.));
#19970=CARTESIAN_POINT('',(22.,-0.75,0.85));
#19971=CARTESIAN_POINT('',(0.,-0.75,0.85));
#19972=CARTESIAN_POINT('',(22.,-0.53,1.));
#19973=CARTESIAN_POINT('',(22.,-0.53,1.));
#19974=CARTESIAN_POINT('',(0.,-0.53,1.));
#19975=CARTESIAN_POINT('Origin',(0.,-0.53,1.15));
#19976=CARTESIAN_POINT('',(0.,-0.53,1.15));
#19977=CARTESIAN_POINT('',(0.,-0.53,1.15));
#19978=CARTESIAN_POINT('',(22.,-0.53,1.15));
#19979=CARTESIAN_POINT('',(22.,-0.53,1.15));
#19980=CARTESIAN_POINT('',(0.,-0.53,1.15));
#19981=CARTESIAN_POINT('Origin',(0.,-0.75,1.3));
#19982=CARTESIAN_POINT('',(0.,-0.75,1.3));
#19983=CARTESIAN_POINT('',(0.,-0.75,1.3));
#19984=CARTESIAN_POINT('',(22.,-0.75,1.3));
#19985=CARTESIAN_POINT('',(22.,-0.75,1.3));
#19986=CARTESIAN_POINT('',(0.,-0.75,1.3));
#19987=CARTESIAN_POINT('Origin',(0.,-0.75,1.5));
#19988=CARTESIAN_POINT('',(0.,-0.75,1.5));
#19989=CARTESIAN_POINT('',(0.,-0.75,1.5));
#19990=CARTESIAN_POINT('',(22.,-0.75,1.5));
#19991=CARTESIAN_POINT('',(22.,-0.75,1.5));
#19992=CARTESIAN_POINT('',(0.,-0.75,1.5));
#19993=CARTESIAN_POINT('Origin',(0.,0.75,1.5));
#19994=CARTESIAN_POINT('',(0.,0.75,1.5));
#19995=CARTESIAN_POINT('',(0.,0.75,1.5));
#19996=CARTESIAN_POINT('',(22.,0.75,1.5));
#19997=CARTESIAN_POINT('',(22.,0.75,1.5));
#19998=CARTESIAN_POINT('',(0.,0.75,1.5));
#19999=CARTESIAN_POINT('Origin',(0.,0.75,1.3));
#20000=CARTESIAN_POINT('',(0.,0.75,1.3));
#20001=CARTESIAN_POINT('',(0.,0.75,1.3));
#20002=CARTESIAN_POINT('',(22.,0.75,1.3));
#20003=CARTESIAN_POINT('',(22.,0.75,1.3));
#20004=CARTESIAN_POINT('',(0.,0.75,1.3));
#20005=CARTESIAN_POINT('Origin',(0.,0.53,1.15));
#20006=CARTESIAN_POINT('',(0.,0.53,1.15));
#20007=CARTESIAN_POINT('',(0.,0.53,1.15));
#20008=CARTESIAN_POINT('',(22.,0.53,1.15));
#20009=CARTESIAN_POINT('',(22.,0.53,1.15));
#20010=CARTESIAN_POINT('',(0.,0.53,1.15));
#20011=CARTESIAN_POINT('Origin',(0.,0.53,1.));
#20012=CARTESIAN_POINT('',(0.,0.53,1.));
#20013=CARTESIAN_POINT('',(0.,0.53,1.));
#20014=CARTESIAN_POINT('',(22.,0.53,1.));
#20015=CARTESIAN_POINT('',(22.,0.53,1.));
#20016=CARTESIAN_POINT('',(0.,0.53,1.));
#20017=CARTESIAN_POINT('Origin',(0.,0.75,0.85));
#20018=CARTESIAN_POINT('',(0.,0.75,0.85));
#20019=CARTESIAN_POINT('',(0.,0.75,0.85));
#20020=CARTESIAN_POINT('',(22.,0.75,0.85));
#20021=CARTESIAN_POINT('',(22.,0.75,0.85));
#20022=CARTESIAN_POINT('',(0.,0.75,0.85));
#20023=CARTESIAN_POINT('Origin',(0.,0.75,0.));
#20024=CARTESIAN_POINT('',(0.,0.75,0.));
#20025=CARTESIAN_POINT('',(0.,0.75,0.));
#20026=CARTESIAN_POINT('',(22.,0.75,0.));
#20027=CARTESIAN_POINT('',(22.,0.75,0.));
#20028=CARTESIAN_POINT('',(0.,0.75,0.));
#20029=CARTESIAN_POINT('Origin',(0.,-0.75,0.));
#20030=CARTESIAN_POINT('',(0.,-0.75,0.));
#20031=CARTESIAN_POINT('',(0.,-0.75,0.));
#20032=CARTESIAN_POINT('',(22.,-0.75,0.));
#20033=CARTESIAN_POINT('',(22.,-0.75,0.));
#20034=CARTESIAN_POINT('',(0.,-0.75,0.));
#20035=CARTESIAN_POINT('Origin',(0.,-0.75,0.85));
#20036=CARTESIAN_POINT('',(0.,-0.75,0.85));
#20037=CARTESIAN_POINT('',(22.,-0.75,0.85));
#20038=CARTESIAN_POINT('Origin',(22.,0.,0.75));
#20039=CARTESIAN_POINT('Origin',(0.,0.,0.75));
#57796=UNCERTAINTY_MEASURE_WITH_UNIT(LENGTH_MEASURE(0.001),#57901,
'DISTANCE_ACCURACY_VALUE',
'Maximum model space distance between geometric entities at asserted c
onnectivities');
#57841=UNCERTAINTY_MEASURE_WITH_UNIT(LENGTH_MEASURE(0.001),#57901,
'DISTANCE_ACCURACY_VALUE',
'Maximum model space distance between geometric entities at asserted c
onnectivities');
#57855=(
GEOMETRIC_REPRESENTATION_CONTEXT(3)
GLOBAL_UNCERTAINTY_ASSIGNED_CONTEXT((#57796))
GLOBAL_UNIT_ASSIGNED_CONTEXT((#57901,#57903,#57904))
REPRESENTATION_CONTEXT('','3D')
);
#57900=(
GEOMETRIC_REPRESENTATION_CONTEXT(3)
GLOBAL_UNCERTAINTY_ASSIGNED_CONTEXT((#57841))
GLOBAL_UNIT_ASSIGNED_CONTEXT((#57901,#57903,#57904))
REPRESENTATION_CONTEXT('','3D')
);
#57901=(
LENGTH_UNIT()
NAMED_UNIT(*)
SI_UNIT(.CENTI.,.METRE.)
);
#57903=(
NAMED_UNIT(*)
PLANE_ANGLE_UNIT()
SI_UNIT($,.RADIAN.)
);
#57904=(
NAMED_UNIT(*)
SI_UNIT($,.STERADIAN.)
SOLID_ANGLE_UNIT()
);
#57918=SHAPE_DEFINITION_REPRESENTATION(#57976,#58122);
#57976=PRODUCT_DEFINITION_SHAPE('',$,#58181);
#58122=SHAPE_REPRESENTATION('',(#14453),#57855);
#58167=PRODUCT_DEFINITION_CONTEXT('part definition',#58343,'design');
#58181=PRODUCT_DEFINITION('Linear Guide Rail - 15 mm, 220 mm Long',
'Linear Guide Rail - 15 mm, 220 mm Long',#58239,#58167);
#58239=PRODUCT_DEFINITION_FORMATION('',$,#58358);
#58343=APPLICATION_CONTEXT(
'Core Data for Automotive Mechanical Design Process');
#58344=PRODUCT_CONTEXT('part definition',#58343,'mechanical');
#58358=PRODUCT('Linear Guide Rail - 15 mm, 220 mm Long',
'Linear Guide Rail - 15 mm, 220 mm Long',
'Linear Guide Rail - 15 mm, 220 mm Long',(#58344));
#58452=COLOUR_RGB('Sky Blue',0.24,0.69,0.87);
#58453=FILL_AREA_STYLE_COLOUR('',#58452);
#58454=FILL_AREA_STYLE('',(#58453));
#58455=SURFACE_STYLE_FILL_AREA(#58454);
#58456=SURFACE_SIDE_STYLE('',(#58455));
#58457=SURFACE_STYLE_USAGE(.BOTH.,#58456);
#58458=PRESENTATION_STYLE_ASSIGNMENT((#58457));
ENDSEC;
END-ISO-10303-21;
